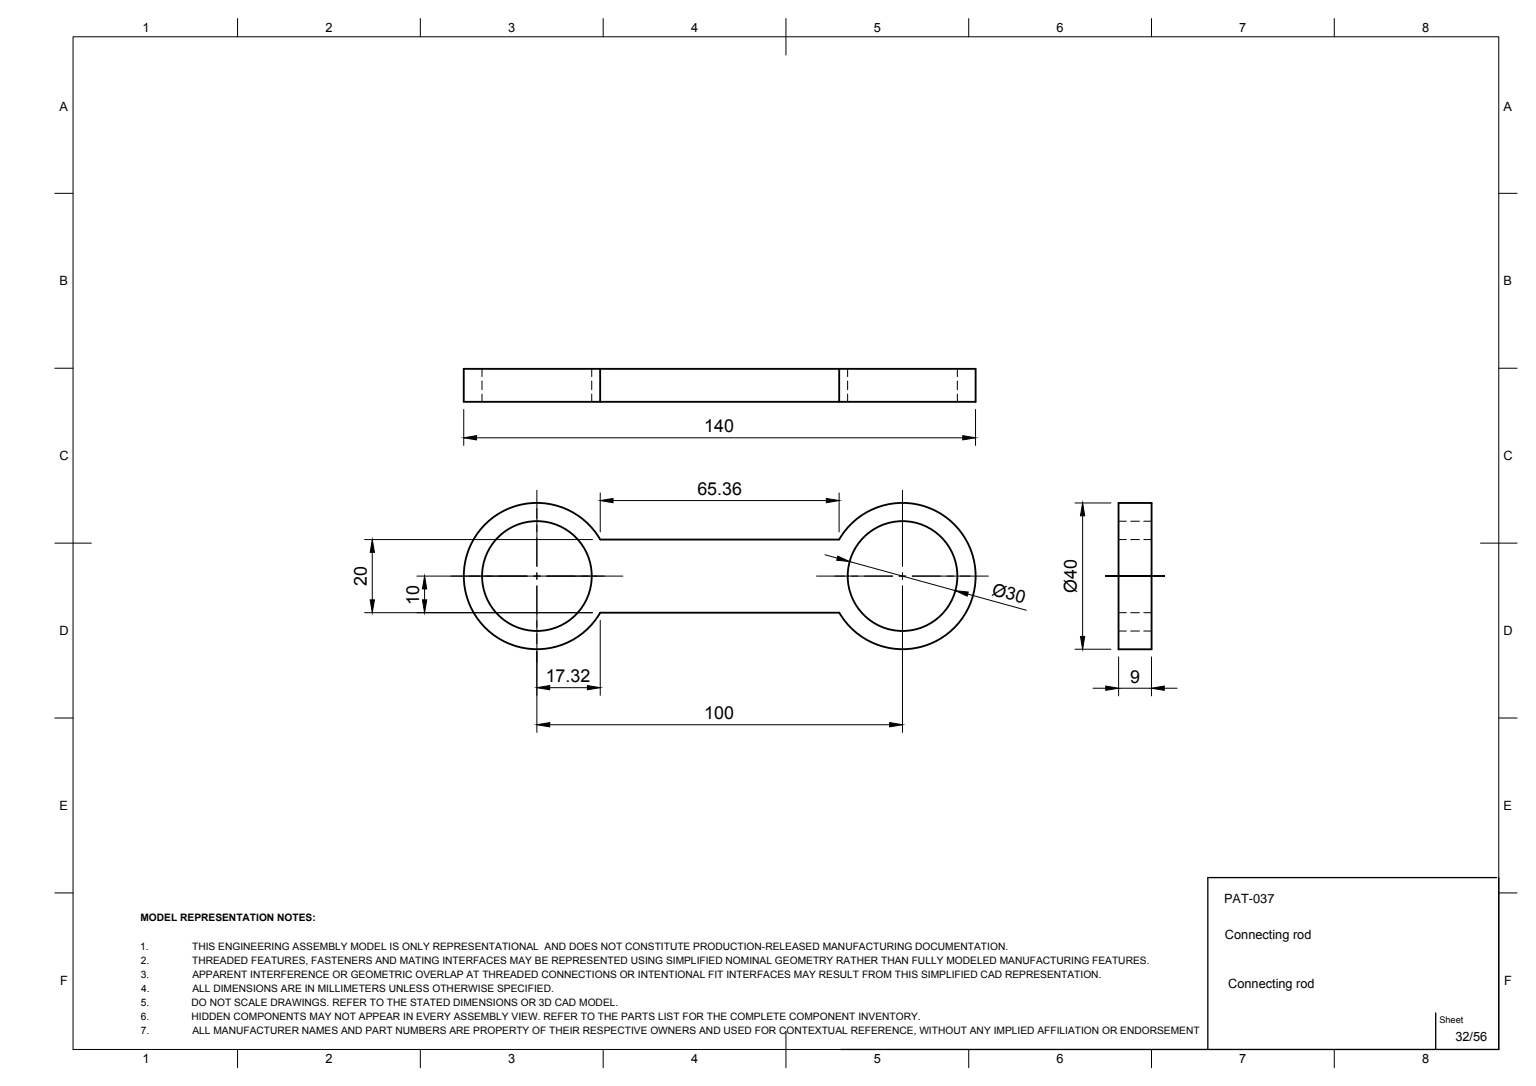
ISO-10303-21;
HEADER;
/* Generated by software containing ST-Developer
 * from STEP Tools, Inc. (www.steptools.com) 
 */

FILE_DESCRIPTION(
/* description */ ('Flywheel Crank-Slider'),
/* implementation_level */ '2;1');

FILE_NAME(
/* name */ 'Connecting rod.step',
/* time_stamp */ '2026-10-28T03:23:13-07:00',
/* author */ (''),
/* organization */ (''),
/* preprocessor_version */ 'ST-DEVELOPER v20.2',
/* originating_system */ 'Autodesk Translation Framework v15.17.0.0',
/* authorisation */ '');

FILE_SCHEMA (('AUTOMOTIVE_DESIGN { 1 0 10303 214 3 1 1 }'));
ENDSEC;

DATA;
#10=MECHANICAL_DESIGN_GEOMETRIC_PRESENTATION_REPRESENTATION('',(#701),#17322);
#596=SHAPE_REPRESENTATION_RELATIONSHIP('SRR','None',#17595,#648);
#648=ADVANCED_BREP_SHAPE_REPRESENTATION('',(#758),#17299);
#701=STYLED_ITEM('',(#17931),#758);
#758=MANIFOLD_SOLID_BREP('Body1',#9083);
#931=FACE_BOUND('',#2363,.T.);
#932=FACE_BOUND('',#2364,.T.);
#933=FACE_BOUND('',#2369,.T.);
#934=FACE_BOUND('',#2370,.T.);
#1230=PLANE('',#10350);
#1231=PLANE('',#10352);
#1232=PLANE('',#10355);
#1233=PLANE('',#10356);
#1678=FACE_OUTER_BOUND('',#2359,.T.);
#1679=FACE_OUTER_BOUND('',#2360,.T.);
#1680=FACE_OUTER_BOUND('',#2361,.T.);
#1681=FACE_OUTER_BOUND('',#2362,.T.);
#1682=FACE_OUTER_BOUND('',#2365,.T.);
#1683=FACE_OUTER_BOUND('',#2366,.T.);
#1684=FACE_OUTER_BOUND('',#2367,.T.);
#1685=FACE_OUTER_BOUND('',#2368,.T.);
#2359=EDGE_LOOP('',(#7614,#7615,#7616,#7617));
#2360=EDGE_LOOP('',(#7618,#7619,#7620,#7621));
#2361=EDGE_LOOP('',(#7622,#7623,#7624,#7625));
#2362=EDGE_LOOP('',(#7626,#7627,#7628,#7629));
#2363=EDGE_LOOP('',(#7630));
#2364=EDGE_LOOP('',(#7631));
#2365=EDGE_LOOP('',(#7632,#7633,#7634,#7635));
#2366=EDGE_LOOP('',(#7636,#7637,#7638,#7639));
#2367=EDGE_LOOP('',(#7640,#7641,#7642,#7643));
#2368=EDGE_LOOP('',(#7644,#7645,#7646,#7647));
#2369=EDGE_LOOP('',(#7648));
#2370=EDGE_LOOP('',(#7649));
#3068=LINE('',#15954,#3679);
#3069=LINE('',#15960,#3680);
#3070=LINE('',#15965,#3681);
#3071=LINE('',#15969,#3682);
#3072=LINE('',#15973,#3683);
#3073=LINE('',#15976,#3684);
#3074=LINE('',#15979,#3685);
#3075=LINE('',#15980,#3686);
#3076=LINE('',#15983,#3687);
#3077=LINE('',#15986,#3688);
#3679=VECTOR('',#12598,1.5);
#3680=VECTOR('',#12605,1.5);
#3681=VECTOR('',#12610,1.);
#3682=VECTOR('',#12613,1.);
#3683=VECTOR('',#12618,1.);
#3684=VECTOR('',#12621,1.);
#3685=VECTOR('',#12624,1.);
#3686=VECTOR('',#12625,1.);
#3687=VECTOR('',#12628,1.);
#3688=VECTOR('',#12633,1.);
#4096=CIRCLE('',#10342,1.5);
#4097=CIRCLE('',#10343,1.5);
#4098=CIRCLE('',#10345,1.5);
#4099=CIRCLE('',#10346,1.5);
#4100=CIRCLE('',#10348,2.);
#4101=CIRCLE('',#10349,2.);
#4102=CIRCLE('',#10351,2.);
#4103=CIRCLE('',#10354,2.);
#4771=VERTEX_POINT('',#15951);
#4772=VERTEX_POINT('',#15953);
#4773=VERTEX_POINT('',#15957);
#4774=VERTEX_POINT('',#15959);
#4775=VERTEX_POINT('',#15963);
#4776=VERTEX_POINT('',#15964);
#4777=VERTEX_POINT('',#15966);
#4778=VERTEX_POINT('',#15968);
#4779=VERTEX_POINT('',#15972);
#4780=VERTEX_POINT('',#15974);
#4781=VERTEX_POINT('',#15978);
#4782=VERTEX_POINT('',#15982);
#5764=EDGE_CURVE('',#4771,#4771,#4096,.T.);
#5765=EDGE_CURVE('',#4771,#4772,#3068,.T.);
#5766=EDGE_CURVE('',#4772,#4772,#4097,.T.);
#5767=EDGE_CURVE('',#4773,#4773,#4098,.T.);
#5768=EDGE_CURVE('',#4773,#4774,#3069,.T.);
#5769=EDGE_CURVE('',#4774,#4774,#4099,.T.);
#5770=EDGE_CURVE('',#4775,#4776,#3070,.T.);
#5771=EDGE_CURVE('',#4775,#4777,#4100,.T.);
#5772=EDGE_CURVE('',#4778,#4777,#3071,.T.);
#5773=EDGE_CURVE('',#4776,#4778,#4101,.T.);
#5774=EDGE_CURVE('',#4778,#4779,#3072,.T.);
#5775=EDGE_CURVE('',#4779,#4780,#4102,.T.);
#5776=EDGE_CURVE('',#4780,#4776,#3073,.T.);
#5777=EDGE_CURVE('',#4781,#4777,#3074,.T.);
#5778=EDGE_CURVE('',#4781,#4779,#3075,.T.);
#5779=EDGE_CURVE('',#4780,#4782,#3076,.T.);
#5780=EDGE_CURVE('',#4781,#4782,#4103,.T.);
#5781=EDGE_CURVE('',#4775,#4782,#3077,.T.);
#7614=ORIENTED_EDGE('',*,*,#5764,.F.);
#7615=ORIENTED_EDGE('',*,*,#5765,.T.);
#7616=ORIENTED_EDGE('',*,*,#5766,.F.);
#7617=ORIENTED_EDGE('',*,*,#5765,.F.);
#7618=ORIENTED_EDGE('',*,*,#5767,.F.);
#7619=ORIENTED_EDGE('',*,*,#5768,.T.);
#7620=ORIENTED_EDGE('',*,*,#5769,.F.);
#7621=ORIENTED_EDGE('',*,*,#5768,.F.);
#7622=ORIENTED_EDGE('',*,*,#5770,.F.);
#7623=ORIENTED_EDGE('',*,*,#5771,.T.);
#7624=ORIENTED_EDGE('',*,*,#5772,.F.);
#7625=ORIENTED_EDGE('',*,*,#5773,.F.);
#7626=ORIENTED_EDGE('',*,*,#5773,.T.);
#7627=ORIENTED_EDGE('',*,*,#5774,.T.);
#7628=ORIENTED_EDGE('',*,*,#5775,.T.);
#7629=ORIENTED_EDGE('',*,*,#5776,.T.);
#7630=ORIENTED_EDGE('',*,*,#5766,.T.);
#7631=ORIENTED_EDGE('',*,*,#5769,.T.);
#7632=ORIENTED_EDGE('',*,*,#5772,.T.);
#7633=ORIENTED_EDGE('',*,*,#5777,.F.);
#7634=ORIENTED_EDGE('',*,*,#5778,.T.);
#7635=ORIENTED_EDGE('',*,*,#5774,.F.);
#7636=ORIENTED_EDGE('',*,*,#5779,.F.);
#7637=ORIENTED_EDGE('',*,*,#5775,.F.);
#7638=ORIENTED_EDGE('',*,*,#5778,.F.);
#7639=ORIENTED_EDGE('',*,*,#5780,.T.);
#7640=ORIENTED_EDGE('',*,*,#5770,.T.);
#7641=ORIENTED_EDGE('',*,*,#5776,.F.);
#7642=ORIENTED_EDGE('',*,*,#5779,.T.);
#7643=ORIENTED_EDGE('',*,*,#5781,.F.);
#7644=ORIENTED_EDGE('',*,*,#5781,.T.);
#7645=ORIENTED_EDGE('',*,*,#5780,.F.);
#7646=ORIENTED_EDGE('',*,*,#5777,.T.);
#7647=ORIENTED_EDGE('',*,*,#5771,.F.);
#7648=ORIENTED_EDGE('',*,*,#5764,.T.);
#7649=ORIENTED_EDGE('',*,*,#5767,.T.);
#8449=CYLINDRICAL_SURFACE('',#10341,1.5);
#8450=CYLINDRICAL_SURFACE('',#10344,1.5);
#8451=CYLINDRICAL_SURFACE('',#10347,2.);
#8452=CYLINDRICAL_SURFACE('',#10353,2.);
#8869=ADVANCED_FACE('',(#1678),#8449,.F.);
#8870=ADVANCED_FACE('',(#1679),#8450,.F.);
#8871=ADVANCED_FACE('',(#1680),#8451,.T.);
#8872=ADVANCED_FACE('',(#1681,#931,#932),#1230,.T.);
#8873=ADVANCED_FACE('',(#1682),#1231,.T.);
#8874=ADVANCED_FACE('',(#1683),#8452,.T.);
#8875=ADVANCED_FACE('',(#1684),#1232,.T.);
#8876=ADVANCED_FACE('',(#1685,#933,#934),#1233,.F.);
#9083=CLOSED_SHELL('',(#8869,#8870,#8871,#8872,#8873,#8874,#8875,#8876));
#10340=AXIS2_PLACEMENT_3D('',#15949,#12592,#12593);
#10341=AXIS2_PLACEMENT_3D('',#15950,#12594,#12595);
#10342=AXIS2_PLACEMENT_3D('',#15952,#12596,#12597);
#10343=AXIS2_PLACEMENT_3D('',#15955,#12599,#12600);
#10344=AXIS2_PLACEMENT_3D('',#15956,#12601,#12602);
#10345=AXIS2_PLACEMENT_3D('',#15958,#12603,#12604);
#10346=AXIS2_PLACEMENT_3D('',#15961,#12606,#12607);
#10347=AXIS2_PLACEMENT_3D('',#15962,#12608,#12609);
#10348=AXIS2_PLACEMENT_3D('',#15967,#12611,#12612);
#10349=AXIS2_PLACEMENT_3D('',#15970,#12614,#12615);
#10350=AXIS2_PLACEMENT_3D('',#15971,#12616,#12617);
#10351=AXIS2_PLACEMENT_3D('',#15975,#12619,#12620);
#10352=AXIS2_PLACEMENT_3D('',#15977,#12622,#12623);
#10353=AXIS2_PLACEMENT_3D('',#15981,#12626,#12627);
#10354=AXIS2_PLACEMENT_3D('',#15984,#12629,#12630);
#10355=AXIS2_PLACEMENT_3D('',#15985,#12631,#12632);
#10356=AXIS2_PLACEMENT_3D('',#15987,#12634,#12635);
#12592=DIRECTION('axis',(0.,0.,1.));
#12593=DIRECTION('refdir',(1.,0.,0.));
#12594=DIRECTION('center_axis',(0.,1.,0.));
#12595=DIRECTION('ref_axis',(1.,0.,0.));
#12596=DIRECTION('center_axis',(0.,1.,0.));
#12597=DIRECTION('ref_axis',(1.,0.,0.));
#12598=DIRECTION('',(0.,1.,0.));
#12599=DIRECTION('center_axis',(0.,-1.,0.));
#12600=DIRECTION('ref_axis',(1.,0.,0.));
#12601=DIRECTION('center_axis',(0.,1.,0.));
#12602=DIRECTION('ref_axis',(1.,0.,0.));
#12603=DIRECTION('center_axis',(0.,1.,0.));
#12604=DIRECTION('ref_axis',(1.,0.,0.));
#12605=DIRECTION('',(0.,1.,0.));
#12606=DIRECTION('center_axis',(0.,-1.,0.));
#12607=DIRECTION('ref_axis',(1.,0.,0.));
#12608=DIRECTION('center_axis',(0.,1.,0.));
#12609=DIRECTION('ref_axis',(1.,0.,0.));
#12610=DIRECTION('',(0.,1.,0.));
#12611=DIRECTION('center_axis',(0.,1.,0.));
#12612=DIRECTION('ref_axis',(1.,0.,0.));
#12613=DIRECTION('',(0.,-1.,0.));
#12614=DIRECTION('center_axis',(0.,1.,0.));
#12615=DIRECTION('ref_axis',(1.,0.,0.));
#12616=DIRECTION('center_axis',(0.,1.,0.));
#12617=DIRECTION('ref_axis',(0.,0.,1.));
#12618=DIRECTION('',(-1.,0.,0.));
#12619=DIRECTION('center_axis',(0.,1.,0.));
#12620=DIRECTION('ref_axis',(1.,0.,0.));
#12621=DIRECTION('',(1.,0.,0.));
#12622=DIRECTION('center_axis',(0.,0.,-1.));
#12623=DIRECTION('ref_axis',(-1.,0.,0.));
#12624=DIRECTION('',(1.,0.,0.));
#12625=DIRECTION('',(0.,1.,0.));
#12626=DIRECTION('center_axis',(0.,1.,0.));
#12627=DIRECTION('ref_axis',(-1.,0.,1.22464679914735E-16));
#12628=DIRECTION('',(0.,-1.,0.));
#12629=DIRECTION('center_axis',(0.,1.,0.));
#12630=DIRECTION('ref_axis',(1.,0.,0.));
#12631=DIRECTION('center_axis',(0.,0.,1.));
#12632=DIRECTION('ref_axis',(1.,0.,0.));
#12633=DIRECTION('',(-1.,0.,0.));
#12634=DIRECTION('center_axis',(0.,1.,0.));
#12635=DIRECTION('ref_axis',(1.,0.,0.));
#15949=CARTESIAN_POINT('',(0.,0.,0.));
#15950=CARTESIAN_POINT('Origin',(2.,2.4,10.));
#15951=CARTESIAN_POINT('',(0.5,2.5,10.));
#15952=CARTESIAN_POINT('Origin',(2.,2.5,10.));
#15953=CARTESIAN_POINT('',(0.5,3.4,10.));
#15954=CARTESIAN_POINT('',(0.5,2.4,10.));
#15955=CARTESIAN_POINT('Origin',(2.,3.4,10.));
#15956=CARTESIAN_POINT('Origin',(12.,2.4,10.));
#15957=CARTESIAN_POINT('',(10.5,2.5,10.));
#15958=CARTESIAN_POINT('Origin',(12.,2.5,10.));
#15959=CARTESIAN_POINT('',(10.5,3.4,10.));
#15960=CARTESIAN_POINT('',(10.5,2.4,10.));
#15961=CARTESIAN_POINT('Origin',(12.,3.4,10.));
#15962=CARTESIAN_POINT('Origin',(12.,2.5,10.));
#15963=CARTESIAN_POINT('',(10.2679491924311,2.5,11.));
#15964=CARTESIAN_POINT('',(10.2679491924311,3.4,11.));
#15965=CARTESIAN_POINT('',(10.2679491924311,2.5,11.));
#15966=CARTESIAN_POINT('',(10.2679491924311,2.5,9.));
#15967=CARTESIAN_POINT('Origin',(12.,2.5,10.));
#15968=CARTESIAN_POINT('',(10.2679491924311,3.4,9.));
#15969=CARTESIAN_POINT('',(10.2679491924311,2.5,9.));
#15970=CARTESIAN_POINT('Origin',(12.,3.4,10.));
#15971=CARTESIAN_POINT('Origin',(7.,3.4,10.));
#15972=CARTESIAN_POINT('',(3.73205080756888,3.4,9.));
#15973=CARTESIAN_POINT('',(2.,3.4,9.));
#15974=CARTESIAN_POINT('',(3.73205080756888,3.4,11.));
#15975=CARTESIAN_POINT('Origin',(2.,3.4,10.));
#15976=CARTESIAN_POINT('',(12.,3.4,11.));
#15977=CARTESIAN_POINT('Origin',(12.,2.5,9.));
#15978=CARTESIAN_POINT('',(3.73205080756888,2.5,9.));
#15979=CARTESIAN_POINT('',(2.,2.5,9.));
#15980=CARTESIAN_POINT('',(3.73205080756888,2.5,9.));
#15981=CARTESIAN_POINT('Origin',(2.,2.5,10.));
#15982=CARTESIAN_POINT('',(3.73205080756888,2.5,11.));
#15983=CARTESIAN_POINT('',(3.73205080756888,2.5,11.));
#15984=CARTESIAN_POINT('Origin',(2.,2.5,10.));
#15985=CARTESIAN_POINT('Origin',(2.,2.5,11.));
#15986=CARTESIAN_POINT('',(12.,2.5,11.));
#15987=CARTESIAN_POINT('Origin',(7.,2.5,10.));
#17238=UNCERTAINTY_MEASURE_WITH_UNIT(LENGTH_MEASURE(0.001),#17323,
'DISTANCE_ACCURACY_VALUE',
'Maximum model space distance between geometric entities at asserted c
onnectivities');
#17261=UNCERTAINTY_MEASURE_WITH_UNIT(LENGTH_MEASURE(0.001),#17323,
'DISTANCE_ACCURACY_VALUE',
'Maximum model space distance between geometric entities at asserted c
onnectivities');
#17299=(
GEOMETRIC_REPRESENTATION_CONTEXT(3)
GLOBAL_UNCERTAINTY_ASSIGNED_CONTEXT((#17238))
GLOBAL_UNIT_ASSIGNED_CONTEXT((#17323,#17325,#17326))
REPRESENTATION_CONTEXT('','3D')
);
#17322=(
GEOMETRIC_REPRESENTATION_CONTEXT(3)
GLOBAL_UNCERTAINTY_ASSIGNED_CONTEXT((#17261))
GLOBAL_UNIT_ASSIGNED_CONTEXT((#17323,#17325,#17326))
REPRESENTATION_CONTEXT('','3D')
);
#17323=(
LENGTH_UNIT()
NAMED_UNIT(*)
SI_UNIT(.CENTI.,.METRE.)
);
#17325=(
NAMED_UNIT(*)
PLANE_ANGLE_UNIT()
SI_UNIT($,.RADIAN.)
);
#17326=(
NAMED_UNIT(*)
SI_UNIT($,.STERADIAN.)
SOLID_ANGLE_UNIT()
);
#17364=SHAPE_DEFINITION_REPRESENTATION(#17426,#17595);
#17426=PRODUCT_DEFINITION_SHAPE('',$,#17656);
#17595=SHAPE_REPRESENTATION('',(#10340),#17299);
#17618=PRODUCT_DEFINITION_CONTEXT('part definition',#17800,'design');
#17656=PRODUCT_DEFINITION('Connecting rod','Connecting rod',#17716,#17618);
#17716=PRODUCT_DEFINITION_FORMATION('',$,#17839);
#17800=APPLICATION_CONTEXT(
'Core Data for Automotive Mechanical Design Process');
#17801=PRODUCT_CONTEXT('part definition',#17800,'mechanical');
#17839=PRODUCT('Connecting rod','Connecting rod','Connecting rod',(#17801));
#17925=COLOUR_RGB('Grey',0.48,0.52,0.57);
#17926=FILL_AREA_STYLE_COLOUR('',#17925);
#17927=FILL_AREA_STYLE('',(#17926));
#17928=SURFACE_STYLE_FILL_AREA(#17927);
#17929=SURFACE_SIDE_STYLE('',(#17928));
#17930=SURFACE_STYLE_USAGE(.BOTH.,#17929);
#17931=PRESENTATION_STYLE_ASSIGNMENT((#17930));
ENDSEC;
END-ISO-10303-21;
